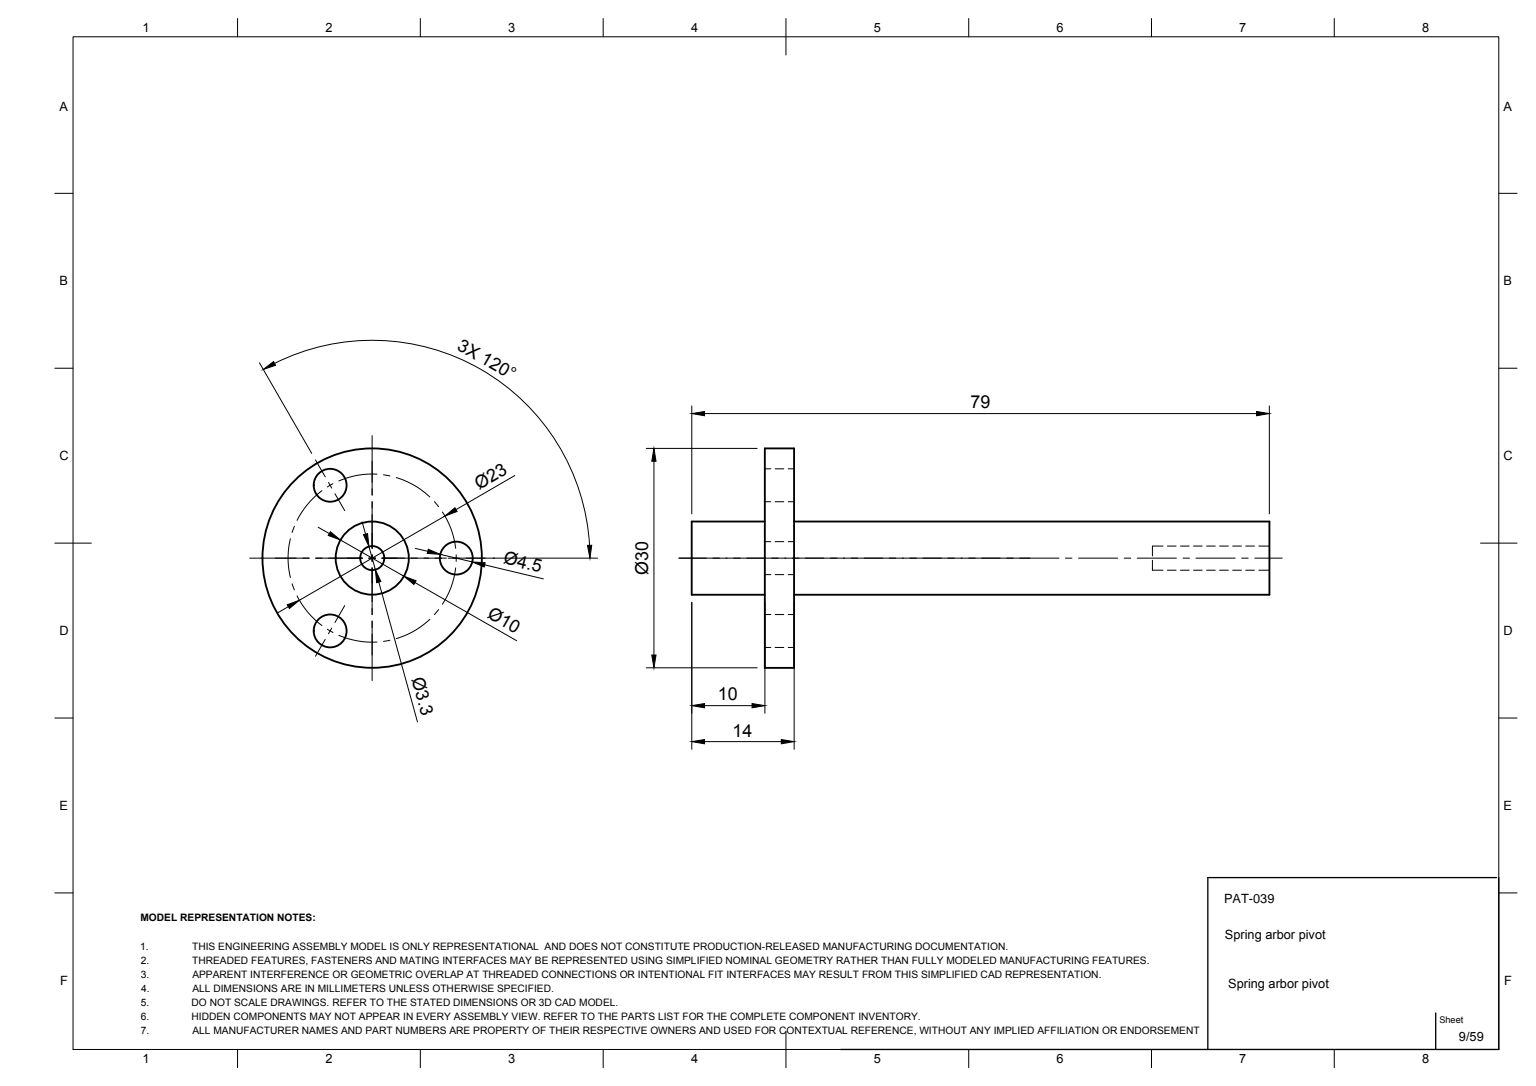
ISO-10303-21;
HEADER;
/* Generated by software containing ST-Developer
 * from STEP Tools, Inc. (www.steptools.com) 
 */

FILE_DESCRIPTION(
/* description */ ('Four-bar parallelogram arm'),
/* implementation_level */ '2;1');

FILE_NAME(
/* name */ 'Spring arbor pivot.step',
/* time_stamp */ '2026-10-28T03:24:55-07:00',
/* author */ (''),
/* organization */ (''),
/* preprocessor_version */ 'ST-DEVELOPER v20.2',
/* originating_system */ 'Autodesk Translation Framework v15.17.0.0',
/* authorisation */ '');

FILE_SCHEMA (('AUTOMOTIVE_DESIGN { 1 0 10303 214 3 1 1 }'));
ENDSEC;

DATA;
#10=MECHANICAL_DESIGN_GEOMETRIC_PRESENTATION_REPRESENTATION('',(#626),#14512);
#526=SHAPE_REPRESENTATION_RELATIONSHIP('SRR','None',#14747,#576);
#576=ADVANCED_BREP_SHAPE_REPRESENTATION('',(#684),#14462);
#626=STYLED_ITEM('',(#15087),#684);
#684=MANIFOLD_SOLID_BREP('Body1',#7330);
#768=FACE_BOUND('',#1706,.T.);
#769=FACE_BOUND('',#1707,.T.);
#770=FACE_BOUND('',#1708,.T.);
#771=FACE_BOUND('',#1709,.T.);
#772=FACE_BOUND('',#1711,.T.);
#773=FACE_BOUND('',#1712,.T.);
#774=FACE_BOUND('',#1713,.T.);
#775=FACE_BOUND('',#1714,.T.);
#776=FACE_BOUND('',#1720,.T.);
#1035=PLANE('',#8028);
#1036=PLANE('',#8038);
#1037=PLANE('',#8041);
#1038=PLANE('',#8049);
#1039=PLANE('',#8050);
#1247=FACE_OUTER_BOUND('',#1700,.T.);
#1248=FACE_OUTER_BOUND('',#1701,.T.);
#1249=FACE_OUTER_BOUND('',#1702,.T.);
#1250=FACE_OUTER_BOUND('',#1703,.T.);
#1251=FACE_OUTER_BOUND('',#1704,.T.);
#1252=FACE_OUTER_BOUND('',#1705,.T.);
#1253=FACE_OUTER_BOUND('',#1710,.T.);
#1254=FACE_OUTER_BOUND('',#1715,.T.);
#1255=FACE_OUTER_BOUND('',#1716,.T.);
#1256=FACE_OUTER_BOUND('',#1717,.T.);
#1257=FACE_OUTER_BOUND('',#1718,.T.);
#1258=FACE_OUTER_BOUND('',#1719,.T.);
#1700=EDGE_LOOP('',(#5210,#5211,#5212,#5213));
#1701=EDGE_LOOP('',(#5214));
#1702=EDGE_LOOP('',(#5215,#5216,#5217,#5218));
#1703=EDGE_LOOP('',(#5219,#5220,#5221,#5222));
#1704=EDGE_LOOP('',(#5223,#5224,#5225,#5226));
#1705=EDGE_LOOP('',(#5227));
#1706=EDGE_LOOP('',(#5228));
#1707=EDGE_LOOP('',(#5229));
#1708=EDGE_LOOP('',(#5230));
#1709=EDGE_LOOP('',(#5231));
#1710=EDGE_LOOP('',(#5232));
#1711=EDGE_LOOP('',(#5233));
#1712=EDGE_LOOP('',(#5234));
#1713=EDGE_LOOP('',(#5235));
#1714=EDGE_LOOP('',(#5236));
#1715=EDGE_LOOP('',(#5237,#5238,#5239,#5240));
#1716=EDGE_LOOP('',(#5241,#5242,#5243,#5244));
#1717=EDGE_LOOP('',(#5245,#5246,#5247,#5248));
#1718=EDGE_LOOP('',(#5249));
#1719=EDGE_LOOP('',(#5250));
#1720=EDGE_LOOP('',(#5251));
#2389=LINE('',#11670,#2783);
#2390=LINE('',#11677,#2784);
#2391=LINE('',#11683,#2785);
#2392=LINE('',#11689,#2786);
#2393=LINE('',#11702,#2787);
#2394=LINE('',#11705,#2788);
#2395=LINE('',#11710,#2789);
#2783=VECTOR('',#9225,0.165);
#2784=VECTOR('',#9234,0.225);
#2785=VECTOR('',#9241,0.225);
#2786=VECTOR('',#9248,0.225);
#2787=VECTOR('',#9265,1.5);
#2788=VECTOR('',#9268,0.5);
#2789=VECTOR('',#9275,0.5);
#3134=CIRCLE('',#8026,0.165);
#3135=CIRCLE('',#8027,0.165);
#3136=CIRCLE('',#8030,0.225);
#3137=CIRCLE('',#8031,0.225);
#3138=CIRCLE('',#8033,0.225);
#3139=CIRCLE('',#8034,0.225);
#3140=CIRCLE('',#8036,0.225);
#3141=CIRCLE('',#8037,0.225);
#3142=CIRCLE('',#8039,1.5);
#3143=CIRCLE('',#8040,0.5);
#3144=CIRCLE('',#8042,1.5);
#3145=CIRCLE('',#8043,0.5);
#3146=CIRCLE('',#8046,0.5);
#3147=CIRCLE('',#8048,0.5);
#3619=VERTEX_POINT('',#11667);
#3620=VERTEX_POINT('',#11669);
#3621=VERTEX_POINT('',#11674);
#3622=VERTEX_POINT('',#11676);
#3623=VERTEX_POINT('',#11680);
#3624=VERTEX_POINT('',#11682);
#3625=VERTEX_POINT('',#11686);
#3626=VERTEX_POINT('',#11688);
#3627=VERTEX_POINT('',#11692);
#3628=VERTEX_POINT('',#11694);
#3629=VERTEX_POINT('',#11697);
#3630=VERTEX_POINT('',#11699);
#3631=VERTEX_POINT('',#11704);
#3632=VERTEX_POINT('',#11708);
#4236=EDGE_CURVE('',#3619,#3619,#3134,.T.);
#4237=EDGE_CURVE('',#3619,#3620,#2389,.T.);
#4238=EDGE_CURVE('',#3620,#3620,#3135,.T.);
#4239=EDGE_CURVE('',#3621,#3621,#3136,.T.);
#4240=EDGE_CURVE('',#3621,#3622,#2390,.T.);
#4241=EDGE_CURVE('',#3622,#3622,#3137,.T.);
#4242=EDGE_CURVE('',#3623,#3623,#3138,.T.);
#4243=EDGE_CURVE('',#3623,#3624,#2391,.T.);
#4244=EDGE_CURVE('',#3624,#3624,#3139,.T.);
#4245=EDGE_CURVE('',#3625,#3625,#3140,.T.);
#4246=EDGE_CURVE('',#3625,#3626,#2392,.T.);
#4247=EDGE_CURVE('',#3626,#3626,#3141,.T.);
#4248=EDGE_CURVE('',#3627,#3627,#3142,.T.);
#4249=EDGE_CURVE('',#3628,#3628,#3143,.T.);
#4250=EDGE_CURVE('',#3629,#3629,#3144,.T.);
#4251=EDGE_CURVE('',#3630,#3630,#3145,.T.);
#4252=EDGE_CURVE('',#3627,#3629,#2393,.T.);
#4253=EDGE_CURVE('',#3630,#3631,#2394,.T.);
#4254=EDGE_CURVE('',#3631,#3631,#3146,.T.);
#4255=EDGE_CURVE('',#3632,#3632,#3147,.T.);
#4256=EDGE_CURVE('',#3632,#3628,#2395,.T.);
#5210=ORIENTED_EDGE('',*,*,#4236,.F.);
#5211=ORIENTED_EDGE('',*,*,#4237,.T.);
#5212=ORIENTED_EDGE('',*,*,#4238,.T.);
#5213=ORIENTED_EDGE('',*,*,#4237,.F.);
#5214=ORIENTED_EDGE('',*,*,#4238,.F.);
#5215=ORIENTED_EDGE('',*,*,#4239,.F.);
#5216=ORIENTED_EDGE('',*,*,#4240,.T.);
#5217=ORIENTED_EDGE('',*,*,#4241,.F.);
#5218=ORIENTED_EDGE('',*,*,#4240,.F.);
#5219=ORIENTED_EDGE('',*,*,#4242,.F.);
#5220=ORIENTED_EDGE('',*,*,#4243,.T.);
#5221=ORIENTED_EDGE('',*,*,#4244,.F.);
#5222=ORIENTED_EDGE('',*,*,#4243,.F.);
#5223=ORIENTED_EDGE('',*,*,#4245,.F.);
#5224=ORIENTED_EDGE('',*,*,#4246,.T.);
#5225=ORIENTED_EDGE('',*,*,#4247,.F.);
#5226=ORIENTED_EDGE('',*,*,#4246,.F.);
#5227=ORIENTED_EDGE('',*,*,#4248,.T.);
#5228=ORIENTED_EDGE('',*,*,#4241,.T.);
#5229=ORIENTED_EDGE('',*,*,#4244,.T.);
#5230=ORIENTED_EDGE('',*,*,#4247,.T.);
#5231=ORIENTED_EDGE('',*,*,#4249,.F.);
#5232=ORIENTED_EDGE('',*,*,#4250,.F.);
#5233=ORIENTED_EDGE('',*,*,#4239,.T.);
#5234=ORIENTED_EDGE('',*,*,#4242,.T.);
#5235=ORIENTED_EDGE('',*,*,#4245,.T.);
#5236=ORIENTED_EDGE('',*,*,#4251,.F.);
#5237=ORIENTED_EDGE('',*,*,#4248,.F.);
#5238=ORIENTED_EDGE('',*,*,#4252,.T.);
#5239=ORIENTED_EDGE('',*,*,#4250,.T.);
#5240=ORIENTED_EDGE('',*,*,#4252,.F.);
#5241=ORIENTED_EDGE('',*,*,#4251,.T.);
#5242=ORIENTED_EDGE('',*,*,#4253,.T.);
#5243=ORIENTED_EDGE('',*,*,#4254,.T.);
#5244=ORIENTED_EDGE('',*,*,#4253,.F.);
#5245=ORIENTED_EDGE('',*,*,#4255,.F.);
#5246=ORIENTED_EDGE('',*,*,#4256,.T.);
#5247=ORIENTED_EDGE('',*,*,#4249,.T.);
#5248=ORIENTED_EDGE('',*,*,#4256,.F.);
#5249=ORIENTED_EDGE('',*,*,#4255,.T.);
#5250=ORIENTED_EDGE('',*,*,#4254,.F.);
#5251=ORIENTED_EDGE('',*,*,#4236,.T.);
#6731=CYLINDRICAL_SURFACE('',#8025,0.165);
#6732=CYLINDRICAL_SURFACE('',#8029,0.225);
#6733=CYLINDRICAL_SURFACE('',#8032,0.225);
#6734=CYLINDRICAL_SURFACE('',#8035,0.225);
#6735=CYLINDRICAL_SURFACE('',#8044,1.5);
#6736=CYLINDRICAL_SURFACE('',#8045,0.5);
#6737=CYLINDRICAL_SURFACE('',#8047,0.5);
#6952=ADVANCED_FACE('',(#1247),#6731,.F.);
#6953=ADVANCED_FACE('',(#1248),#1035,.F.);
#6954=ADVANCED_FACE('',(#1249),#6732,.F.);
#6955=ADVANCED_FACE('',(#1250),#6733,.F.);
#6956=ADVANCED_FACE('',(#1251),#6734,.F.);
#6957=ADVANCED_FACE('',(#1252,#768,#769,#770,#771),#1036,.T.);
#6958=ADVANCED_FACE('',(#1253,#772,#773,#774,#775),#1037,.F.);
#6959=ADVANCED_FACE('',(#1254),#6735,.T.);
#6960=ADVANCED_FACE('',(#1255),#6736,.T.);
#6961=ADVANCED_FACE('',(#1256),#6737,.T.);
#6962=ADVANCED_FACE('',(#1257),#1038,.T.);
#6963=ADVANCED_FACE('',(#1258,#776),#1039,.F.);
#7330=CLOSED_SHELL('',(#6952,#6953,#6954,#6955,#6956,#6957,#6958,#6959,
#6960,#6961,#6962,#6963));
#8024=AXIS2_PLACEMENT_3D('',#11665,#9219,#9220);
#8025=AXIS2_PLACEMENT_3D('',#11666,#9221,#9222);
#8026=AXIS2_PLACEMENT_3D('',#11668,#9223,#9224);
#8027=AXIS2_PLACEMENT_3D('',#11671,#9226,#9227);
#8028=AXIS2_PLACEMENT_3D('',#11672,#9228,#9229);
#8029=AXIS2_PLACEMENT_3D('',#11673,#9230,#9231);
#8030=AXIS2_PLACEMENT_3D('',#11675,#9232,#9233);
#8031=AXIS2_PLACEMENT_3D('',#11678,#9235,#9236);
#8032=AXIS2_PLACEMENT_3D('',#11679,#9237,#9238);
#8033=AXIS2_PLACEMENT_3D('',#11681,#9239,#9240);
#8034=AXIS2_PLACEMENT_3D('',#11684,#9242,#9243);
#8035=AXIS2_PLACEMENT_3D('',#11685,#9244,#9245);
#8036=AXIS2_PLACEMENT_3D('',#11687,#9246,#9247);
#8037=AXIS2_PLACEMENT_3D('',#11690,#9249,#9250);
#8038=AXIS2_PLACEMENT_3D('',#11691,#9251,#9252);
#8039=AXIS2_PLACEMENT_3D('',#11693,#9253,#9254);
#8040=AXIS2_PLACEMENT_3D('',#11695,#9255,#9256);
#8041=AXIS2_PLACEMENT_3D('',#11696,#9257,#9258);
#8042=AXIS2_PLACEMENT_3D('',#11698,#9259,#9260);
#8043=AXIS2_PLACEMENT_3D('',#11700,#9261,#9262);
#8044=AXIS2_PLACEMENT_3D('',#11701,#9263,#9264);
#8045=AXIS2_PLACEMENT_3D('',#11703,#9266,#9267);
#8046=AXIS2_PLACEMENT_3D('',#11706,#9269,#9270);
#8047=AXIS2_PLACEMENT_3D('',#11707,#9271,#9272);
#8048=AXIS2_PLACEMENT_3D('',#11709,#9273,#9274);
#8049=AXIS2_PLACEMENT_3D('',#11711,#9276,#9277);
#8050=AXIS2_PLACEMENT_3D('',#11712,#9278,#9279);
#9219=DIRECTION('axis',(0.,0.,1.));
#9220=DIRECTION('refdir',(1.,0.,0.));
#9221=DIRECTION('center_axis',(0.,1.,0.));
#9222=DIRECTION('ref_axis',(1.,0.,0.));
#9223=DIRECTION('center_axis',(0.,1.,0.));
#9224=DIRECTION('ref_axis',(1.,0.,0.));
#9225=DIRECTION('',(0.,1.,0.));
#9226=DIRECTION('center_axis',(0.,1.,0.));
#9227=DIRECTION('ref_axis',(1.,0.,0.));
#9228=DIRECTION('center_axis',(0.,1.,0.));
#9229=DIRECTION('ref_axis',(1.,0.,0.));
#9230=DIRECTION('center_axis',(0.,1.,0.));
#9231=DIRECTION('ref_axis',(1.,0.,0.));
#9232=DIRECTION('center_axis',(0.,1.,0.));
#9233=DIRECTION('ref_axis',(1.,0.,0.));
#9234=DIRECTION('',(0.,1.,0.));
#9235=DIRECTION('center_axis',(0.,-1.,0.));
#9236=DIRECTION('ref_axis',(1.,0.,0.));
#9237=DIRECTION('center_axis',(0.,1.,0.));
#9238=DIRECTION('ref_axis',(1.,0.,0.));
#9239=DIRECTION('center_axis',(0.,1.,0.));
#9240=DIRECTION('ref_axis',(1.,0.,0.));
#9241=DIRECTION('',(0.,1.,0.));
#9242=DIRECTION('center_axis',(0.,-1.,0.));
#9243=DIRECTION('ref_axis',(1.,0.,0.));
#9244=DIRECTION('center_axis',(0.,1.,0.));
#9245=DIRECTION('ref_axis',(1.,0.,0.));
#9246=DIRECTION('center_axis',(0.,1.,0.));
#9247=DIRECTION('ref_axis',(1.,0.,0.));
#9248=DIRECTION('',(0.,1.,0.));
#9249=DIRECTION('center_axis',(0.,-1.,0.));
#9250=DIRECTION('ref_axis',(1.,0.,0.));
#9251=DIRECTION('center_axis',(0.,1.,0.));
#9252=DIRECTION('ref_axis',(1.,0.,0.));
#9253=DIRECTION('center_axis',(0.,1.,0.));
#9254=DIRECTION('ref_axis',(1.,0.,0.));
#9255=DIRECTION('center_axis',(0.,1.,0.));
#9256=DIRECTION('ref_axis',(1.,0.,0.));
#9257=DIRECTION('center_axis',(0.,1.,0.));
#9258=DIRECTION('ref_axis',(1.,0.,0.));
#9259=DIRECTION('center_axis',(0.,1.,0.));
#9260=DIRECTION('ref_axis',(1.,0.,0.));
#9261=DIRECTION('center_axis',(0.,-1.,0.));
#9262=DIRECTION('ref_axis',(1.,0.,0.));
#9263=DIRECTION('center_axis',(0.,1.,0.));
#9264=DIRECTION('ref_axis',(1.,0.,0.));
#9265=DIRECTION('',(0.,-1.,0.));
#9266=DIRECTION('center_axis',(0.,1.,0.));
#9267=DIRECTION('ref_axis',(1.,0.,0.));
#9268=DIRECTION('',(0.,-1.,0.));
#9269=DIRECTION('center_axis',(0.,1.,0.));
#9270=DIRECTION('ref_axis',(1.,0.,0.));
#9271=DIRECTION('center_axis',(0.,1.,0.));
#9272=DIRECTION('ref_axis',(1.,0.,0.));
#9273=DIRECTION('center_axis',(0.,1.,0.));
#9274=DIRECTION('ref_axis',(1.,0.,0.));
#9275=DIRECTION('',(0.,-1.,0.));
#9276=DIRECTION('center_axis',(0.,1.,0.));
#9277=DIRECTION('ref_axis',(1.,0.,0.));
#9278=DIRECTION('center_axis',(0.,1.,0.));
#9279=DIRECTION('ref_axis',(1.,0.,0.));
#11665=CARTESIAN_POINT('',(0.,0.,0.));
#11666=CARTESIAN_POINT('Origin',(0.,-4.1,8.));
#11667=CARTESIAN_POINT('',(-0.165,-4.,8.));
#11668=CARTESIAN_POINT('Origin',(0.,-4.,8.));
#11669=CARTESIAN_POINT('',(-0.165,-2.4,8.));
#11670=CARTESIAN_POINT('',(-0.165,-4.1,8.));
#11671=CARTESIAN_POINT('Origin',(0.,-2.4,8.));
#11672=CARTESIAN_POINT('Origin',(0.,-2.4,8.));
#11673=CARTESIAN_POINT('Origin',(1.15,2.4,8.));
#11674=CARTESIAN_POINT('',(0.925,2.5,8.));
#11675=CARTESIAN_POINT('Origin',(1.15,2.5,8.));
#11676=CARTESIAN_POINT('',(0.925,2.9,8.));
#11677=CARTESIAN_POINT('',(0.925,2.4,8.));
#11678=CARTESIAN_POINT('Origin',(1.15,2.9,8.));
#11679=CARTESIAN_POINT('Origin',(-0.575,2.4,8.9959292143521));
#11680=CARTESIAN_POINT('',(-0.8,2.5,8.9959292143521));
#11681=CARTESIAN_POINT('Origin',(-0.575,2.5,8.9959292143521));
#11682=CARTESIAN_POINT('',(-0.8,2.9,8.9959292143521));
#11683=CARTESIAN_POINT('',(-0.8,2.4,8.9959292143521));
#11684=CARTESIAN_POINT('Origin',(-0.575,2.9,8.9959292143521));
#11685=CARTESIAN_POINT('Origin',(-0.575000000000001,2.4,7.0040707856479));
#11686=CARTESIAN_POINT('',(-0.8,2.5,7.0040707856479));
#11687=CARTESIAN_POINT('Origin',(-0.575000000000001,2.5,7.0040707856479));
#11688=CARTESIAN_POINT('',(-0.8,2.9,7.0040707856479));
#11689=CARTESIAN_POINT('',(-0.8,2.4,7.0040707856479));
#11690=CARTESIAN_POINT('Origin',(-0.575000000000001,2.9,7.0040707856479));
#11691=CARTESIAN_POINT('Origin',(0.,2.9,8.));
#11692=CARTESIAN_POINT('',(-1.5,2.9,8.));
#11693=CARTESIAN_POINT('Origin',(0.,2.9,8.));
#11694=CARTESIAN_POINT('',(-0.5,2.9,8.));
#11695=CARTESIAN_POINT('Origin',(0.,2.9,8.));
#11696=CARTESIAN_POINT('Origin',(0.,2.5,8.));
#11697=CARTESIAN_POINT('',(-1.5,2.5,8.));
#11698=CARTESIAN_POINT('Origin',(0.,2.5,8.));
#11699=CARTESIAN_POINT('',(-0.5,2.5,8.));
#11700=CARTESIAN_POINT('Origin',(0.,2.5,8.));
#11701=CARTESIAN_POINT('Origin',(0.,2.5,8.));
#11702=CARTESIAN_POINT('',(-1.5,2.5,8.));
#11703=CARTESIAN_POINT('Origin',(0.,-4.,8.));
#11704=CARTESIAN_POINT('',(-0.5,-4.,8.));
#11705=CARTESIAN_POINT('',(-0.5,-4.,8.));
#11706=CARTESIAN_POINT('Origin',(0.,-4.,8.));
#11707=CARTESIAN_POINT('Origin',(0.,-4.,8.));
#11708=CARTESIAN_POINT('',(-0.5,3.9,8.));
#11709=CARTESIAN_POINT('Origin',(0.,3.9,8.));
#11710=CARTESIAN_POINT('',(-0.5,-4.,8.));
#11711=CARTESIAN_POINT('Origin',(0.,3.9,8.));
#11712=CARTESIAN_POINT('Origin',(0.,-4.,8.));
#14405=UNCERTAINTY_MEASURE_WITH_UNIT(LENGTH_MEASURE(0.001),#14513,
'DISTANCE_ACCURACY_VALUE',
'Maximum model space distance between geometric entities at asserted c
onnectivities');
#14455=UNCERTAINTY_MEASURE_WITH_UNIT(LENGTH_MEASURE(0.001),#14513,
'DISTANCE_ACCURACY_VALUE',
'Maximum model space distance between geometric entities at asserted c
onnectivities');
#14462=(
GEOMETRIC_REPRESENTATION_CONTEXT(3)
GLOBAL_UNCERTAINTY_ASSIGNED_CONTEXT((#14405))
GLOBAL_UNIT_ASSIGNED_CONTEXT((#14513,#14515,#14516))
REPRESENTATION_CONTEXT('','3D')
);
#14512=(
GEOMETRIC_REPRESENTATION_CONTEXT(3)
GLOBAL_UNCERTAINTY_ASSIGNED_CONTEXT((#14455))
GLOBAL_UNIT_ASSIGNED_CONTEXT((#14513,#14515,#14516))
REPRESENTATION_CONTEXT('','3D')
);
#14513=(
LENGTH_UNIT()
NAMED_UNIT(*)
SI_UNIT(.CENTI.,.METRE.)
);
#14515=(
NAMED_UNIT(*)
PLANE_ANGLE_UNIT()
SI_UNIT($,.RADIAN.)
);
#14516=(
NAMED_UNIT(*)
SI_UNIT($,.STERADIAN.)
SOLID_ANGLE_UNIT()
);
#14523=SHAPE_DEFINITION_REPRESENTATION(#14579,#14747);
#14579=PRODUCT_DEFINITION_SHAPE('',$,#14804);
#14747=SHAPE_REPRESENTATION('',(#8024),#14462);
#14797=PRODUCT_DEFINITION_CONTEXT('part definition',#14967,'design');
#14804=PRODUCT_DEFINITION('Spring arbor pivot','Spring arbor pivot',#14860,
#14797);
#14860=PRODUCT_DEFINITION_FORMATION('',$,#14975);
#14967=APPLICATION_CONTEXT(
'Core Data for Automotive Mechanical Design Process');
#14968=PRODUCT_CONTEXT('part definition',#14967,'mechanical');
#14975=PRODUCT('Spring arbor pivot','Spring arbor pivot',
'Spring arbor pivot',(#14968));
#15081=COLOUR_RGB('Grey',0.48,0.52,0.57);
#15082=FILL_AREA_STYLE_COLOUR('',#15081);
#15083=FILL_AREA_STYLE('',(#15082));
#15084=SURFACE_STYLE_FILL_AREA(#15083);
#15085=SURFACE_SIDE_STYLE('',(#15084));
#15086=SURFACE_STYLE_USAGE(.BOTH.,#15085);
#15087=PRESENTATION_STYLE_ASSIGNMENT((#15086));
ENDSEC;
END-ISO-10303-21;
